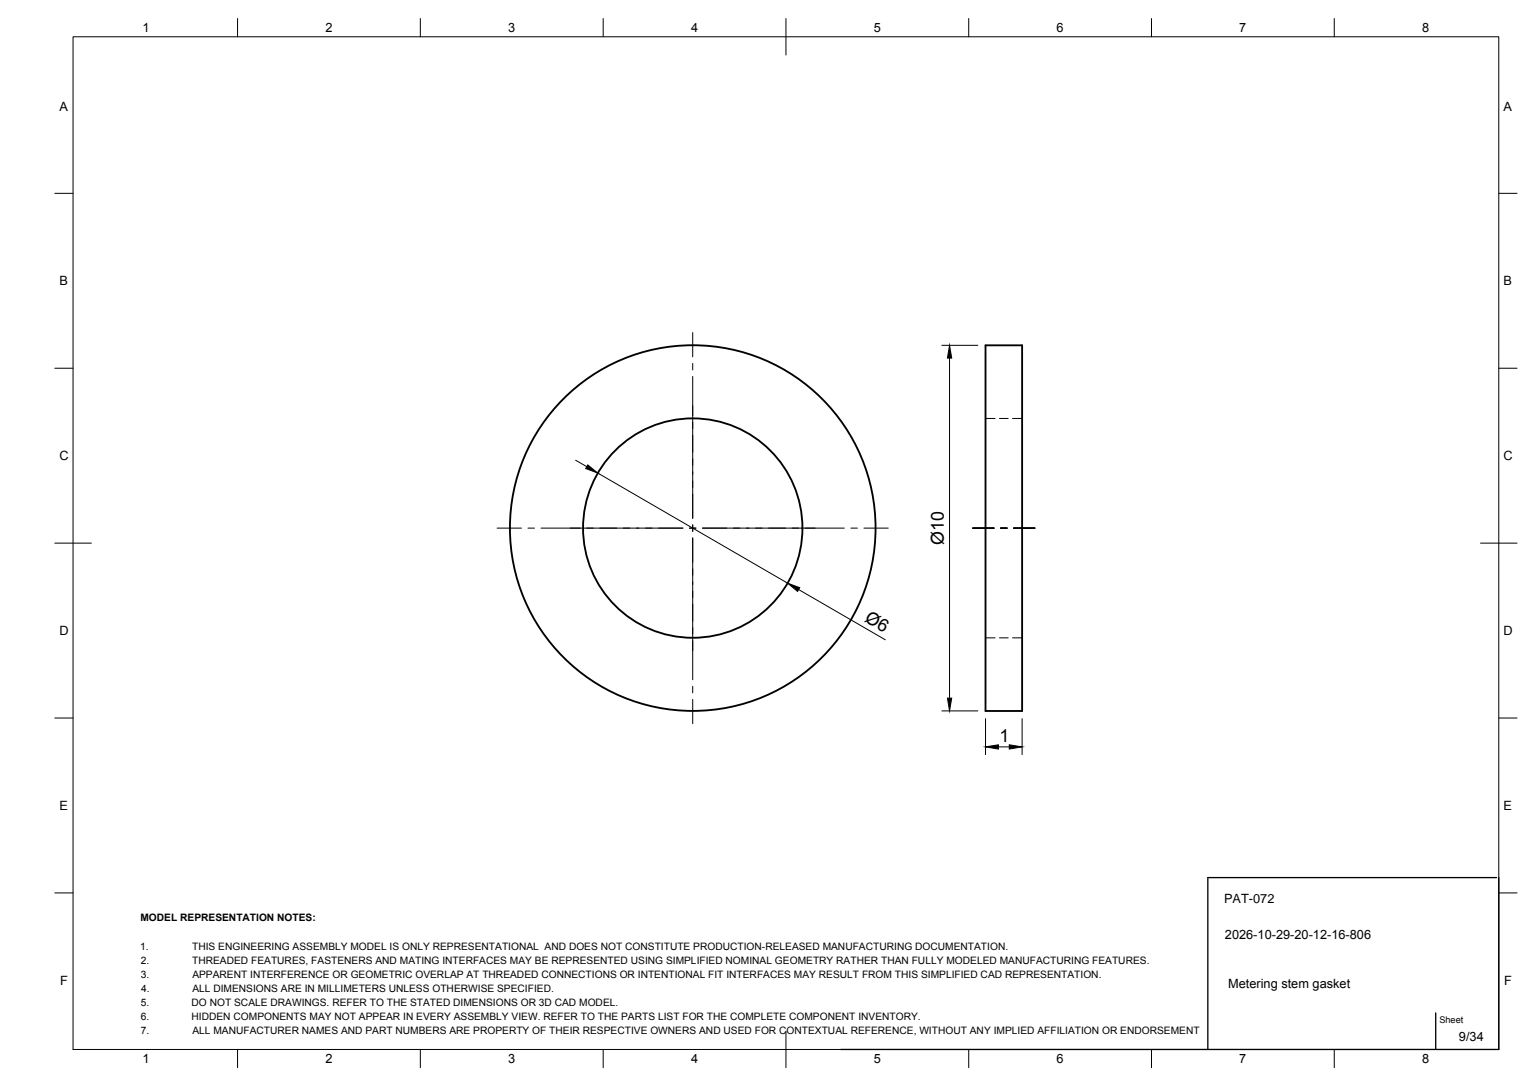
ISO-10303-21;
HEADER;
/* Generated by software containing ST-Developer
 * from STEP Tools, Inc. (www.steptools.com) 
 */

FILE_DESCRIPTION(
/* description */ ('PAT-072'),
/* implementation_level */ '2;1');

FILE_NAME(
/* name */ 'Metering stem gasket.step',
/* time_stamp */ '2026-10-29T20:11:56-07:00',
/* author */ (''),
/* organization */ (''),
/* preprocessor_version */ 'ST-DEVELOPER v20.2',
/* originating_system */ 'Autodesk Translation Framework v15.17.0.0',
/* authorisation */ '');

FILE_SCHEMA (('AUTOMOTIVE_DESIGN { 1 0 10303 214 3 1 1 }'));
ENDSEC;

DATA;
#10=MECHANICAL_DESIGN_GEOMETRIC_PRESENTATION_REPRESENTATION('',(#338),#11432);
#266=SHAPE_REPRESENTATION_RELATIONSHIP('SRR','None',#11570,#302);
#302=ADVANCED_BREP_SHAPE_REPRESENTATION('',(#374),#11401);
#338=STYLED_ITEM('',(#11833),#374);
#374=MANIFOLD_SOLID_BREP('Body1',#6073);
#464=FACE_BOUND('',#1341,.T.);
#465=FACE_BOUND('',#1343,.T.);
#627=PLANE('',#6722);
#628=PLANE('',#6723);
#904=FACE_OUTER_BOUND('',#1338,.T.);
#905=FACE_OUTER_BOUND('',#1339,.T.);
#906=FACE_OUTER_BOUND('',#1340,.T.);
#907=FACE_OUTER_BOUND('',#1342,.T.);
#1338=EDGE_LOOP('',(#4528,#4529,#4530,#4531));
#1339=EDGE_LOOP('',(#4532,#4533,#4534,#4535));
#1340=EDGE_LOOP('',(#4536));
#1341=EDGE_LOOP('',(#4537));
#1342=EDGE_LOOP('',(#4538));
#1343=EDGE_LOOP('',(#4539));
#1815=LINE('',#10031,#2234);
#1816=LINE('',#10037,#2235);
#2234=VECTOR('',#7798,0.3);
#2235=VECTOR('',#7805,0.5);
#2637=CIRCLE('',#6717,0.3);
#2638=CIRCLE('',#6718,0.3);
#2639=CIRCLE('',#6720,0.5);
#2640=CIRCLE('',#6721,0.5);
#2986=VERTEX_POINT('',#10028);
#2987=VERTEX_POINT('',#10030);
#2988=VERTEX_POINT('',#10034);
#2989=VERTEX_POINT('',#10036);
#3553=EDGE_CURVE('',#2986,#2986,#2637,.T.);
#3554=EDGE_CURVE('',#2986,#2987,#1815,.T.);
#3555=EDGE_CURVE('',#2987,#2987,#2638,.T.);
#3556=EDGE_CURVE('',#2988,#2988,#2639,.T.);
#3557=EDGE_CURVE('',#2988,#2989,#1816,.T.);
#3558=EDGE_CURVE('',#2989,#2989,#2640,.T.);
#4528=ORIENTED_EDGE('',*,*,#3553,.F.);
#4529=ORIENTED_EDGE('',*,*,#3554,.T.);
#4530=ORIENTED_EDGE('',*,*,#3555,.T.);
#4531=ORIENTED_EDGE('',*,*,#3554,.F.);
#4532=ORIENTED_EDGE('',*,*,#3556,.F.);
#4533=ORIENTED_EDGE('',*,*,#3557,.T.);
#4534=ORIENTED_EDGE('',*,*,#3558,.T.);
#4535=ORIENTED_EDGE('',*,*,#3557,.F.);
#4536=ORIENTED_EDGE('',*,*,#3556,.T.);
#4537=ORIENTED_EDGE('',*,*,#3553,.T.);
#4538=ORIENTED_EDGE('',*,*,#3558,.F.);
#4539=ORIENTED_EDGE('',*,*,#3555,.F.);
#5609=CYLINDRICAL_SURFACE('',#6716,0.3);
#5610=CYLINDRICAL_SURFACE('',#6719,0.5);
#5803=ADVANCED_FACE('',(#904),#5609,.F.);
#5804=ADVANCED_FACE('',(#905),#5610,.T.);
#5805=ADVANCED_FACE('',(#906,#464),#627,.T.);
#5806=ADVANCED_FACE('',(#907,#465),#628,.F.);
#6073=CLOSED_SHELL('',(#5803,#5804,#5805,#5806));
#6715=AXIS2_PLACEMENT_3D('',#10026,#7792,#7793);
#6716=AXIS2_PLACEMENT_3D('',#10027,#7794,#7795);
#6717=AXIS2_PLACEMENT_3D('',#10029,#7796,#7797);
#6718=AXIS2_PLACEMENT_3D('',#10032,#7799,#7800);
#6719=AXIS2_PLACEMENT_3D('',#10033,#7801,#7802);
#6720=AXIS2_PLACEMENT_3D('',#10035,#7803,#7804);
#6721=AXIS2_PLACEMENT_3D('',#10038,#7806,#7807);
#6722=AXIS2_PLACEMENT_3D('',#10039,#7808,#7809);
#6723=AXIS2_PLACEMENT_3D('',#10040,#7810,#7811);
#7792=DIRECTION('axis',(0.,0.,1.));
#7793=DIRECTION('refdir',(1.,0.,0.));
#7794=DIRECTION('center_axis',(0.,0.,1.));
#7795=DIRECTION('ref_axis',(1.,0.,0.));
#7796=DIRECTION('center_axis',(0.,0.,-1.));
#7797=DIRECTION('ref_axis',(1.,0.,0.));
#7798=DIRECTION('',(0.,0.,-1.));
#7799=DIRECTION('center_axis',(0.,0.,-1.));
#7800=DIRECTION('ref_axis',(1.,0.,0.));
#7801=DIRECTION('center_axis',(0.,0.,1.));
#7802=DIRECTION('ref_axis',(1.,0.,0.));
#7803=DIRECTION('center_axis',(0.,0.,1.));
#7804=DIRECTION('ref_axis',(1.,0.,0.));
#7805=DIRECTION('',(0.,0.,-1.));
#7806=DIRECTION('center_axis',(0.,0.,1.));
#7807=DIRECTION('ref_axis',(1.,0.,0.));
#7808=DIRECTION('center_axis',(0.,0.,1.));
#7809=DIRECTION('ref_axis',(1.,0.,0.));
#7810=DIRECTION('center_axis',(0.,0.,1.));
#7811=DIRECTION('ref_axis',(1.,0.,0.));
#10026=CARTESIAN_POINT('',(0.,0.,0.));
#10027=CARTESIAN_POINT('Origin',(-3.75,1.5,6.));
#10028=CARTESIAN_POINT('',(-4.05,1.5,6.1));
#10029=CARTESIAN_POINT('Origin',(-3.75,1.5,6.1));
#10030=CARTESIAN_POINT('',(-4.05,1.5,6.));
#10031=CARTESIAN_POINT('',(-4.05,1.5,6.));
#10032=CARTESIAN_POINT('Origin',(-3.75,1.5,6.));
#10033=CARTESIAN_POINT('Origin',(-3.75,1.5,6.));
#10034=CARTESIAN_POINT('',(-4.25,1.5,6.1));
#10035=CARTESIAN_POINT('Origin',(-3.75,1.5,6.1));
#10036=CARTESIAN_POINT('',(-4.25,1.5,6.));
#10037=CARTESIAN_POINT('',(-4.25,1.5,6.));
#10038=CARTESIAN_POINT('Origin',(-3.75,1.5,6.));
#10039=CARTESIAN_POINT('Origin',(-3.75,1.5,6.1));
#10040=CARTESIAN_POINT('Origin',(-3.75,1.5,6.));
#11362=UNCERTAINTY_MEASURE_WITH_UNIT(LENGTH_MEASURE(0.001),#11433,
'DISTANCE_ACCURACY_VALUE',
'Maximum model space distance between geometric entities at asserted c
onnectivities');
#11393=UNCERTAINTY_MEASURE_WITH_UNIT(LENGTH_MEASURE(0.001),#11433,
'DISTANCE_ACCURACY_VALUE',
'Maximum model space distance between geometric entities at asserted c
onnectivities');
#11401=(
GEOMETRIC_REPRESENTATION_CONTEXT(3)
GLOBAL_UNCERTAINTY_ASSIGNED_CONTEXT((#11362))
GLOBAL_UNIT_ASSIGNED_CONTEXT((#11433,#11435,#11436))
REPRESENTATION_CONTEXT('','3D')
);
#11432=(
GEOMETRIC_REPRESENTATION_CONTEXT(3)
GLOBAL_UNCERTAINTY_ASSIGNED_CONTEXT((#11393))
GLOBAL_UNIT_ASSIGNED_CONTEXT((#11433,#11435,#11436))
REPRESENTATION_CONTEXT('','3D')
);
#11433=(
LENGTH_UNIT()
NAMED_UNIT(*)
SI_UNIT(.CENTI.,.METRE.)
);
#11435=(
NAMED_UNIT(*)
PLANE_ANGLE_UNIT()
SI_UNIT($,.RADIAN.)
);
#11436=(
NAMED_UNIT(*)
SI_UNIT($,.STERADIAN.)
SOLID_ANGLE_UNIT()
);
#11444=SHAPE_DEFINITION_REPRESENTATION(#11482,#11570);
#11482=PRODUCT_DEFINITION_SHAPE('',$,#11609);
#11570=SHAPE_REPRESENTATION('',(#6715),#11401);
#11601=PRODUCT_DEFINITION_CONTEXT('part definition',#11717,'design');
#11609=PRODUCT_DEFINITION('Metering stem gasket',
'Metering stem gasket',#11647,#11601);
#11647=PRODUCT_DEFINITION_FORMATION('',$,#11726);
#11717=APPLICATION_CONTEXT(
'Core Data for Automotive Mechanical Design Process');
#11718=PRODUCT_CONTEXT('part definition',#11717,'mechanical');
#11726=PRODUCT('Metering stem gasket','Metering stem gasket',
'Metering stem gasket',(#11718));
#11827=COLOUR_RGB('Off White',0.89,0.88,0.83);
#11828=FILL_AREA_STYLE_COLOUR('',#11827);
#11829=FILL_AREA_STYLE('',(#11828));
#11830=SURFACE_STYLE_FILL_AREA(#11829);
#11831=SURFACE_SIDE_STYLE('',(#11830));
#11832=SURFACE_STYLE_USAGE(.BOTH.,#11831);
#11833=PRESENTATION_STYLE_ASSIGNMENT((#11832));
ENDSEC;
END-ISO-10303-21;
